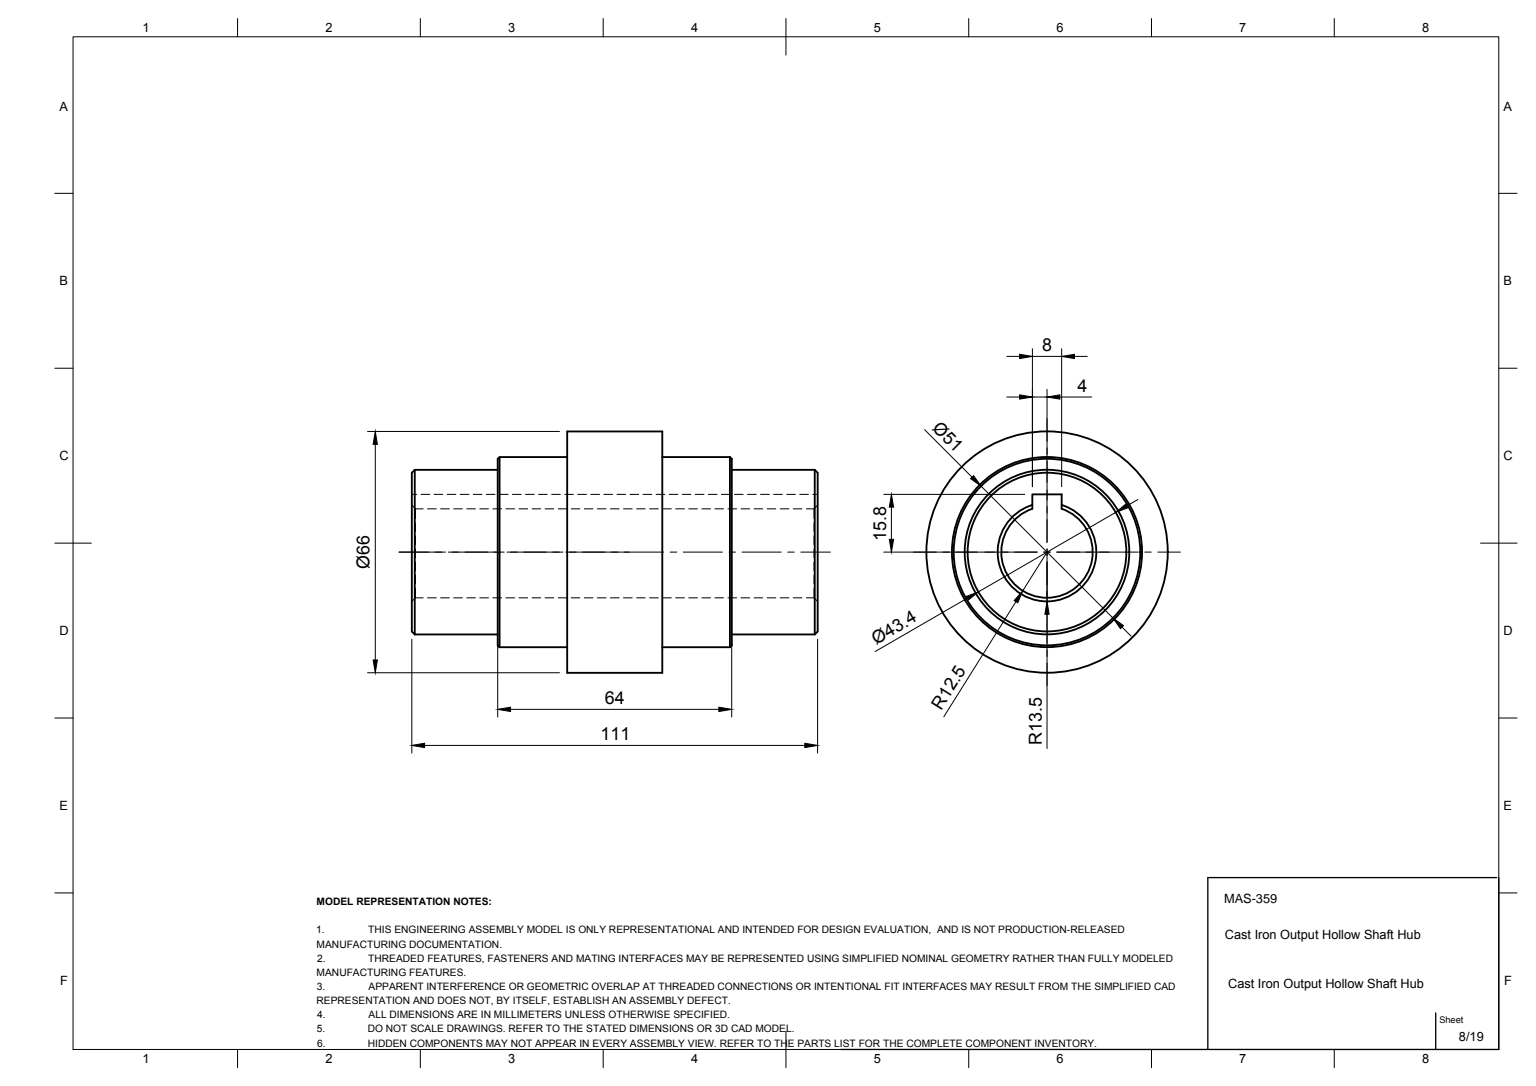
ISO-10303-21;
HEADER;
/* Generated by software containing ST-Developer
 * from STEP Tools, Inc. (www.steptools.com) 
 */

FILE_DESCRIPTION(
/* description */ (''),
/* implementation_level */ '2;1');

FILE_NAME(
/* name */ 'Cast Iron Output Hollow Shaft Hub.step',
/* time_stamp */ '2026-10-15T14:25:16-07:00',
/* author */ (''),
/* organization */ (''),
/* preprocessor_version */ 'ST-DEVELOPER v20.2',
/* originating_system */ 'Autodesk Translation Framework v15.15.0.0',
/* authorisation */ '');

FILE_SCHEMA (('AUTOMOTIVE_DESIGN { 1 0 10303 214 3 1 1 }'));
ENDSEC;

DATA;
#10=MECHANICAL_DESIGN_GEOMETRIC_PRESENTATION_REPRESENTATION('',(#328),#86429);
#262=(
BOUNDED_CURVE()
B_SPLINE_CURVE(2,(#63092,#63093,#63094),.UNSPECIFIED.,.F.,.F.)
B_SPLINE_CURVE_WITH_KNOTS((3,3),(0.,0.145078131153909),.UNSPECIFIED.)
CURVE()
GEOMETRIC_REPRESENTATION_ITEM()
RATIONAL_B_SPLINE_CURVE((1.,1.00081813630177,1.))
REPRESENTATION_ITEM('')
);
#263=(
BOUNDED_CURVE()
B_SPLINE_CURVE(2,(#63097,#63098,#63099),.UNSPECIFIED.,.F.,.F.)
B_SPLINE_CURVE_WITH_KNOTS((3,3),(0.,0.145078131153909),.UNSPECIFIED.)
CURVE()
GEOMETRIC_REPRESENTATION_ITEM()
RATIONAL_B_SPLINE_CURVE((1.,1.00081813630177,1.))
REPRESENTATION_ITEM('')
);
#264=(
BOUNDED_CURVE()
B_SPLINE_CURVE(2,(#63110,#63111,#63112),.UNSPECIFIED.,.F.,.F.)
B_SPLINE_CURVE_WITH_KNOTS((3,3),(0.,0.145078131153909),.UNSPECIFIED.)
CURVE()
GEOMETRIC_REPRESENTATION_ITEM()
RATIONAL_B_SPLINE_CURVE((1.,1.00081813630177,1.))
REPRESENTATION_ITEM('')
);
#265=(
BOUNDED_CURVE()
B_SPLINE_CURVE(2,(#63116,#63117,#63118),.UNSPECIFIED.,.F.,.F.)
B_SPLINE_CURVE_WITH_KNOTS((3,3),(0.,0.145078131153909),.UNSPECIFIED.)
CURVE()
GEOMETRIC_REPRESENTATION_ITEM()
RATIONAL_B_SPLINE_CURVE((1.,1.00081813630177,1.))
REPRESENTATION_ITEM('')
);
#292=SHAPE_REPRESENTATION_RELATIONSHIP('SRR','None',#86507,#310);
#310=ADVANCED_BREP_SHAPE_REPRESENTATION('',(#346),#86416);
#328=STYLED_ITEM('',(#86606),#346);
#346=MANIFOLD_SOLID_BREP('Body1',#15618);
#1297=CONICAL_SURFACE('',#16826,1.3,0.785398163397457);
#1298=CONICAL_SURFACE('',#16828,2.21,0.785398163397443);
#1299=CONICAL_SURFACE('',#16834,2.575,0.785398163397453);
#1300=CONICAL_SURFACE('',#16846,2.575,0.785398163397453);
#1301=CONICAL_SURFACE('',#16852,2.21,0.785398163397443);
#1302=CONICAL_SURFACE('',#16856,1.3,0.785398163397457);
#1507=CYLINDRICAL_SURFACE('',#16830,2.25);
#1508=CYLINDRICAL_SURFACE('',#16836,2.6);
#1509=CYLINDRICAL_SURFACE('',#16840,3.3);
#1510=CYLINDRICAL_SURFACE('',#16844,2.6);
#1511=CYLINDRICAL_SURFACE('',#16850,2.25);
#1512=CYLINDRICAL_SURFACE('',#16858,1.25);
#1706=FACE_BOUND('',#3993,.T.);
#1707=FACE_BOUND('',#3998,.T.);
#1708=FACE_BOUND('',#4002,.T.);
#1709=FACE_BOUND('',#4005,.T.);
#1710=FACE_BOUND('',#4009,.T.);
#1711=FACE_BOUND('',#4013,.T.);
#2198=CIRCLE('',#16824,2.17);
#2199=CIRCLE('',#16825,1.35);
#2200=CIRCLE('',#16827,1.25);
#2201=CIRCLE('',#16829,2.25);
#2202=CIRCLE('',#16831,2.25);
#2203=CIRCLE('',#16833,2.55);
#2204=CIRCLE('',#16835,2.6);
#2205=CIRCLE('',#16837,2.6);
#2206=CIRCLE('',#16839,3.3);
#2207=CIRCLE('',#16841,3.3);
#2208=CIRCLE('',#16843,2.6);
#2209=CIRCLE('',#16845,2.6);
#2210=CIRCLE('',#16847,2.55);
#2211=CIRCLE('',#16849,2.25);
#2212=CIRCLE('',#16851,2.25);
#2213=CIRCLE('',#16853,2.17);
#2214=CIRCLE('',#16855,1.35);
#2215=CIRCLE('',#16857,1.25);
#3013=FACE_OUTER_BOUND('',#3989,.T.);
#3014=FACE_OUTER_BOUND('',#3990,.T.);
#3015=FACE_OUTER_BOUND('',#3991,.T.);
#3016=FACE_OUTER_BOUND('',#3992,.T.);
#3017=FACE_OUTER_BOUND('',#3994,.T.);
#3018=FACE_OUTER_BOUND('',#3995,.T.);
#3019=FACE_OUTER_BOUND('',#3996,.T.);
#3020=FACE_OUTER_BOUND('',#3997,.T.);
#3021=FACE_OUTER_BOUND('',#3999,.T.);
#3022=FACE_OUTER_BOUND('',#4000,.T.);
#3023=FACE_OUTER_BOUND('',#4001,.T.);
#3024=FACE_OUTER_BOUND('',#4003,.T.);
#3025=FACE_OUTER_BOUND('',#4004,.T.);
#3026=FACE_OUTER_BOUND('',#4006,.T.);
#3027=FACE_OUTER_BOUND('',#4007,.T.);
#3028=FACE_OUTER_BOUND('',#4008,.T.);
#3029=FACE_OUTER_BOUND('',#4010,.T.);
#3030=FACE_OUTER_BOUND('',#4011,.T.);
#3031=FACE_OUTER_BOUND('',#4012,.T.);
#3032=FACE_OUTER_BOUND('',#4014,.T.);
#3033=FACE_OUTER_BOUND('',#4015,.T.);
#3989=EDGE_LOOP('',(#13157,#13158,#13159,#13160,#13161,#13162));
#3990=EDGE_LOOP('',(#13163,#13164,#13165,#13166));
#3991=EDGE_LOOP('',(#13167,#13168,#13169,#13170,#13171,#13172));
#3992=EDGE_LOOP('',(#13173));
#3993=EDGE_LOOP('',(#13174,#13175,#13176,#13177));
#3994=EDGE_LOOP('',(#13178,#13179,#13180,#13181));
#3995=EDGE_LOOP('',(#13182,#13183,#13184,#13185));
#3996=EDGE_LOOP('',(#13186,#13187,#13188,#13189));
#3997=EDGE_LOOP('',(#13190));
#3998=EDGE_LOOP('',(#13191));
#3999=EDGE_LOOP('',(#13192,#13193,#13194,#13195));
#4000=EDGE_LOOP('',(#13196,#13197,#13198,#13199));
#4001=EDGE_LOOP('',(#13200));
#4002=EDGE_LOOP('',(#13201));
#4003=EDGE_LOOP('',(#13202,#13203,#13204,#13205));
#4004=EDGE_LOOP('',(#13206));
#4005=EDGE_LOOP('',(#13207));
#4006=EDGE_LOOP('',(#13208,#13209,#13210,#13211));
#4007=EDGE_LOOP('',(#13212,#13213,#13214,#13215));
#4008=EDGE_LOOP('',(#13216));
#4009=EDGE_LOOP('',(#13217));
#4010=EDGE_LOOP('',(#13218,#13219,#13220,#13221));
#4011=EDGE_LOOP('',(#13222,#13223,#13224,#13225));
#4012=EDGE_LOOP('',(#13226));
#4013=EDGE_LOOP('',(#13227,#13228,#13229,#13230));
#4014=EDGE_LOOP('',(#13231,#13232,#13233,#13234));
#4015=EDGE_LOOP('',(#13235,#13236,#13237,#13238));
#4949=LINE('',#63086,#5809);
#4950=LINE('',#63088,#5810);
#4951=LINE('',#63090,#5811);
#4952=LINE('',#63096,#5812);
#4953=LINE('',#63102,#5813);
#4954=LINE('',#63104,#5814);
#4955=LINE('',#63105,#5815);
#4956=LINE('',#63108,#5816);
#4957=LINE('',#63114,#5817);
#4958=LINE('',#63119,#5818);
#4959=LINE('',#63129,#5819);
#4960=LINE('',#63133,#5820);
#4961=LINE('',#63140,#5821);
#4962=LINE('',#63144,#5822);
#4963=LINE('',#63151,#5823);
#4964=LINE('',#63158,#5824);
#4965=LINE('',#63161,#5825);
#4966=LINE('',#63169,#5826);
#4967=LINE('',#63172,#5827);
#5809=VECTOR('',#19936,1.);
#5810=VECTOR('',#19937,1.);
#5811=VECTOR('',#19938,1.);
#5812=VECTOR('',#19939,1.);
#5813=VECTOR('',#19942,1.);
#5814=VECTOR('',#19943,1.);
#5815=VECTOR('',#19944,1.);
#5816=VECTOR('',#19947,1.);
#5817=VECTOR('',#19948,1.);
#5818=VECTOR('',#19949,1.);
#5819=VECTOR('',#19964,2.21);
#5820=VECTOR('',#19969,2.25);
#5821=VECTOR('',#19978,2.575);
#5822=VECTOR('',#19983,2.6);
#5823=VECTOR('',#19992,3.3);
#5824=VECTOR('',#20001,2.6);
#5825=VECTOR('',#20004,2.575);
#5826=VECTOR('',#20015,2.25);
#5827=VECTOR('',#20018,2.21);
#7082=VERTEX_POINT('',#63084);
#7083=VERTEX_POINT('',#63085);
#7084=VERTEX_POINT('',#63087);
#7085=VERTEX_POINT('',#63089);
#7086=VERTEX_POINT('',#63091);
#7087=VERTEX_POINT('',#63095);
#7088=VERTEX_POINT('',#63101);
#7089=VERTEX_POINT('',#63103);
#7090=VERTEX_POINT('',#63107);
#7091=VERTEX_POINT('',#63109);
#7092=VERTEX_POINT('',#63113);
#7093=VERTEX_POINT('',#63115);
#7094=VERTEX_POINT('',#63121);
#7095=VERTEX_POINT('',#63127);
#7096=VERTEX_POINT('',#63131);
#7097=VERTEX_POINT('',#63135);
#7098=VERTEX_POINT('',#63138);
#7099=VERTEX_POINT('',#63142);
#7100=VERTEX_POINT('',#63146);
#7101=VERTEX_POINT('',#63149);
#7102=VERTEX_POINT('',#63153);
#7103=VERTEX_POINT('',#63156);
#7104=VERTEX_POINT('',#63160);
#7105=VERTEX_POINT('',#63164);
#7106=VERTEX_POINT('',#63167);
#7107=VERTEX_POINT('',#63171);
#9200=EDGE_CURVE('',#7082,#7083,#4949,.T.);
#9201=EDGE_CURVE('',#7082,#7084,#4950,.T.);
#9202=EDGE_CURVE('',#7085,#7084,#4951,.T.);
#9203=EDGE_CURVE('',#7086,#7085,#262,.T.);
#9204=EDGE_CURVE('',#7087,#7086,#4952,.T.);
#9205=EDGE_CURVE('',#7083,#7087,#263,.T.);
#9206=EDGE_CURVE('',#7088,#7082,#4953,.T.);
#9207=EDGE_CURVE('',#7089,#7088,#4954,.T.);
#9208=EDGE_CURVE('',#7084,#7089,#4955,.T.);
#9209=EDGE_CURVE('',#7090,#7088,#4956,.T.);
#9210=EDGE_CURVE('',#7091,#7090,#264,.T.);
#9211=EDGE_CURVE('',#7092,#7091,#4957,.T.);
#9212=EDGE_CURVE('',#7093,#7092,#265,.T.);
#9213=EDGE_CURVE('',#7089,#7093,#4958,.T.);
#9214=EDGE_CURVE('',#7094,#7094,#2198,.T.);
#9215=EDGE_CURVE('',#7083,#7090,#2199,.T.);
#9216=EDGE_CURVE('',#7087,#7091,#2200,.T.);
#9217=EDGE_CURVE('',#7095,#7095,#2201,.T.);
#9218=EDGE_CURVE('',#7095,#7094,#4959,.T.);
#9219=EDGE_CURVE('',#7096,#7096,#2202,.T.);
#9220=EDGE_CURVE('',#7096,#7095,#4960,.T.);
#9221=EDGE_CURVE('',#7097,#7097,#2203,.T.);
#9222=EDGE_CURVE('',#7098,#7098,#2204,.T.);
#9223=EDGE_CURVE('',#7098,#7097,#4961,.T.);
#9224=EDGE_CURVE('',#7099,#7099,#2205,.T.);
#9225=EDGE_CURVE('',#7099,#7098,#4962,.T.);
#9226=EDGE_CURVE('',#7100,#7100,#2206,.T.);
#9227=EDGE_CURVE('',#7101,#7101,#2207,.T.);
#9228=EDGE_CURVE('',#7101,#7100,#4963,.T.);
#9229=EDGE_CURVE('',#7102,#7102,#2208,.T.);
#9230=EDGE_CURVE('',#7103,#7103,#2209,.T.);
#9231=EDGE_CURVE('',#7103,#7102,#4964,.T.);
#9232=EDGE_CURVE('',#7103,#7104,#4965,.T.);
#9233=EDGE_CURVE('',#7104,#7104,#2210,.T.);
#9234=EDGE_CURVE('',#7105,#7105,#2211,.T.);
#9235=EDGE_CURVE('',#7106,#7106,#2212,.T.);
#9236=EDGE_CURVE('',#7106,#7105,#4966,.T.);
#9237=EDGE_CURVE('',#7106,#7107,#4967,.T.);
#9238=EDGE_CURVE('',#7107,#7107,#2213,.T.);
#9239=EDGE_CURVE('',#7085,#7093,#2214,.T.);
#9240=EDGE_CURVE('',#7086,#7092,#2215,.T.);
#13157=ORIENTED_EDGE('',*,*,#9200,.F.);
#13158=ORIENTED_EDGE('',*,*,#9201,.T.);
#13159=ORIENTED_EDGE('',*,*,#9202,.F.);
#13160=ORIENTED_EDGE('',*,*,#9203,.F.);
#13161=ORIENTED_EDGE('',*,*,#9204,.F.);
#13162=ORIENTED_EDGE('',*,*,#9205,.F.);
#13163=ORIENTED_EDGE('',*,*,#9206,.F.);
#13164=ORIENTED_EDGE('',*,*,#9207,.F.);
#13165=ORIENTED_EDGE('',*,*,#9208,.F.);
#13166=ORIENTED_EDGE('',*,*,#9201,.F.);
#13167=ORIENTED_EDGE('',*,*,#9209,.F.);
#13168=ORIENTED_EDGE('',*,*,#9210,.F.);
#13169=ORIENTED_EDGE('',*,*,#9211,.F.);
#13170=ORIENTED_EDGE('',*,*,#9212,.F.);
#13171=ORIENTED_EDGE('',*,*,#9213,.F.);
#13172=ORIENTED_EDGE('',*,*,#9207,.T.);
#13173=ORIENTED_EDGE('',*,*,#9214,.F.);
#13174=ORIENTED_EDGE('',*,*,#9209,.T.);
#13175=ORIENTED_EDGE('',*,*,#9206,.T.);
#13176=ORIENTED_EDGE('',*,*,#9200,.T.);
#13177=ORIENTED_EDGE('',*,*,#9215,.T.);
#13178=ORIENTED_EDGE('',*,*,#9210,.T.);
#13179=ORIENTED_EDGE('',*,*,#9215,.F.);
#13180=ORIENTED_EDGE('',*,*,#9205,.T.);
#13181=ORIENTED_EDGE('',*,*,#9216,.T.);
#13182=ORIENTED_EDGE('',*,*,#9217,.F.);
#13183=ORIENTED_EDGE('',*,*,#9218,.T.);
#13184=ORIENTED_EDGE('',*,*,#9214,.T.);
#13185=ORIENTED_EDGE('',*,*,#9218,.F.);
#13186=ORIENTED_EDGE('',*,*,#9219,.F.);
#13187=ORIENTED_EDGE('',*,*,#9220,.T.);
#13188=ORIENTED_EDGE('',*,*,#9217,.T.);
#13189=ORIENTED_EDGE('',*,*,#9220,.F.);
#13190=ORIENTED_EDGE('',*,*,#9221,.F.);
#13191=ORIENTED_EDGE('',*,*,#9219,.T.);
#13192=ORIENTED_EDGE('',*,*,#9222,.F.);
#13193=ORIENTED_EDGE('',*,*,#9223,.T.);
#13194=ORIENTED_EDGE('',*,*,#9221,.T.);
#13195=ORIENTED_EDGE('',*,*,#9223,.F.);
#13196=ORIENTED_EDGE('',*,*,#9224,.F.);
#13197=ORIENTED_EDGE('',*,*,#9225,.T.);
#13198=ORIENTED_EDGE('',*,*,#9222,.T.);
#13199=ORIENTED_EDGE('',*,*,#9225,.F.);
#13200=ORIENTED_EDGE('',*,*,#9226,.F.);
#13201=ORIENTED_EDGE('',*,*,#9224,.T.);
#13202=ORIENTED_EDGE('',*,*,#9227,.F.);
#13203=ORIENTED_EDGE('',*,*,#9228,.T.);
#13204=ORIENTED_EDGE('',*,*,#9226,.T.);
#13205=ORIENTED_EDGE('',*,*,#9228,.F.);
#13206=ORIENTED_EDGE('',*,*,#9227,.T.);
#13207=ORIENTED_EDGE('',*,*,#9229,.F.);
#13208=ORIENTED_EDGE('',*,*,#9230,.F.);
#13209=ORIENTED_EDGE('',*,*,#9231,.T.);
#13210=ORIENTED_EDGE('',*,*,#9229,.T.);
#13211=ORIENTED_EDGE('',*,*,#9231,.F.);
#13212=ORIENTED_EDGE('',*,*,#9230,.T.);
#13213=ORIENTED_EDGE('',*,*,#9232,.T.);
#13214=ORIENTED_EDGE('',*,*,#9233,.F.);
#13215=ORIENTED_EDGE('',*,*,#9232,.F.);
#13216=ORIENTED_EDGE('',*,*,#9233,.T.);
#13217=ORIENTED_EDGE('',*,*,#9234,.F.);
#13218=ORIENTED_EDGE('',*,*,#9235,.F.);
#13219=ORIENTED_EDGE('',*,*,#9236,.T.);
#13220=ORIENTED_EDGE('',*,*,#9234,.T.);
#13221=ORIENTED_EDGE('',*,*,#9236,.F.);
#13222=ORIENTED_EDGE('',*,*,#9235,.T.);
#13223=ORIENTED_EDGE('',*,*,#9237,.T.);
#13224=ORIENTED_EDGE('',*,*,#9238,.F.);
#13225=ORIENTED_EDGE('',*,*,#9237,.F.);
#13226=ORIENTED_EDGE('',*,*,#9238,.T.);
#13227=ORIENTED_EDGE('',*,*,#9213,.T.);
#13228=ORIENTED_EDGE('',*,*,#9239,.F.);
#13229=ORIENTED_EDGE('',*,*,#9202,.T.);
#13230=ORIENTED_EDGE('',*,*,#9208,.T.);
#13231=ORIENTED_EDGE('',*,*,#9212,.T.);
#13232=ORIENTED_EDGE('',*,*,#9240,.F.);
#13233=ORIENTED_EDGE('',*,*,#9203,.T.);
#13234=ORIENTED_EDGE('',*,*,#9239,.T.);
#13235=ORIENTED_EDGE('',*,*,#9211,.T.);
#13236=ORIENTED_EDGE('',*,*,#9216,.F.);
#13237=ORIENTED_EDGE('',*,*,#9204,.T.);
#13238=ORIENTED_EDGE('',*,*,#9240,.T.);
#14656=PLANE('',#16820);
#14657=PLANE('',#16821);
#14658=PLANE('',#16822);
#14659=PLANE('',#16823);
#14660=PLANE('',#16832);
#14661=PLANE('',#16838);
#14662=PLANE('',#16842);
#14663=PLANE('',#16848);
#14664=PLANE('',#16854);
#15369=ADVANCED_FACE('',(#3013),#14656,.F.);
#15370=ADVANCED_FACE('',(#3014),#14657,.F.);
#15371=ADVANCED_FACE('',(#3015),#14658,.F.);
#15372=ADVANCED_FACE('',(#3016,#1706),#14659,.T.);
#15373=ADVANCED_FACE('',(#3017),#1297,.F.);
#15374=ADVANCED_FACE('',(#3018),#1298,.T.);
#15375=ADVANCED_FACE('',(#3019),#1507,.T.);
#15376=ADVANCED_FACE('',(#3020,#1707),#14660,.T.);
#15377=ADVANCED_FACE('',(#3021),#1299,.T.);
#15378=ADVANCED_FACE('',(#3022),#1508,.T.);
#15379=ADVANCED_FACE('',(#3023,#1708),#14661,.T.);
#15380=ADVANCED_FACE('',(#3024),#1509,.T.);
#15381=ADVANCED_FACE('',(#3025,#1709),#14662,.T.);
#15382=ADVANCED_FACE('',(#3026),#1510,.T.);
#15383=ADVANCED_FACE('',(#3027),#1300,.T.);
#15384=ADVANCED_FACE('',(#3028,#1710),#14663,.T.);
#15385=ADVANCED_FACE('',(#3029),#1511,.T.);
#15386=ADVANCED_FACE('',(#3030),#1301,.T.);
#15387=ADVANCED_FACE('',(#3031,#1711),#14664,.T.);
#15388=ADVANCED_FACE('',(#3032),#1302,.F.);
#15389=ADVANCED_FACE('',(#3033),#1512,.F.);
#15618=CLOSED_SHELL('',(#15369,#15370,#15371,#15372,#15373,#15374,#15375,
#15376,#15377,#15378,#15379,#15380,#15381,#15382,#15383,#15384,#15385,#15386,
#15387,#15388,#15389));
#16819=AXIS2_PLACEMENT_3D('',#63082,#19932,#19933);
#16820=AXIS2_PLACEMENT_3D('',#63083,#19934,#19935);
#16821=AXIS2_PLACEMENT_3D('',#63100,#19940,#19941);
#16822=AXIS2_PLACEMENT_3D('',#63106,#19945,#19946);
#16823=AXIS2_PLACEMENT_3D('',#63120,#19950,#19951);
#16824=AXIS2_PLACEMENT_3D('',#63122,#19952,#19953);
#16825=AXIS2_PLACEMENT_3D('',#63123,#19954,#19955);
#16826=AXIS2_PLACEMENT_3D('',#63124,#19956,#19957);
#16827=AXIS2_PLACEMENT_3D('',#63125,#19958,#19959);
#16828=AXIS2_PLACEMENT_3D('',#63126,#19960,#19961);
#16829=AXIS2_PLACEMENT_3D('',#63128,#19962,#19963);
#16830=AXIS2_PLACEMENT_3D('',#63130,#19965,#19966);
#16831=AXIS2_PLACEMENT_3D('',#63132,#19967,#19968);
#16832=AXIS2_PLACEMENT_3D('',#63134,#19970,#19971);
#16833=AXIS2_PLACEMENT_3D('',#63136,#19972,#19973);
#16834=AXIS2_PLACEMENT_3D('',#63137,#19974,#19975);
#16835=AXIS2_PLACEMENT_3D('',#63139,#19976,#19977);
#16836=AXIS2_PLACEMENT_3D('',#63141,#19979,#19980);
#16837=AXIS2_PLACEMENT_3D('',#63143,#19981,#19982);
#16838=AXIS2_PLACEMENT_3D('',#63145,#19984,#19985);
#16839=AXIS2_PLACEMENT_3D('',#63147,#19986,#19987);
#16840=AXIS2_PLACEMENT_3D('',#63148,#19988,#19989);
#16841=AXIS2_PLACEMENT_3D('',#63150,#19990,#19991);
#16842=AXIS2_PLACEMENT_3D('',#63152,#19993,#19994);
#16843=AXIS2_PLACEMENT_3D('',#63154,#19995,#19996);
#16844=AXIS2_PLACEMENT_3D('',#63155,#19997,#19998);
#16845=AXIS2_PLACEMENT_3D('',#63157,#19999,#20000);
#16846=AXIS2_PLACEMENT_3D('',#63159,#20002,#20003);
#16847=AXIS2_PLACEMENT_3D('',#63162,#20005,#20006);
#16848=AXIS2_PLACEMENT_3D('',#63163,#20007,#20008);
#16849=AXIS2_PLACEMENT_3D('',#63165,#20009,#20010);
#16850=AXIS2_PLACEMENT_3D('',#63166,#20011,#20012);
#16851=AXIS2_PLACEMENT_3D('',#63168,#20013,#20014);
#16852=AXIS2_PLACEMENT_3D('',#63170,#20016,#20017);
#16853=AXIS2_PLACEMENT_3D('',#63173,#20019,#20020);
#16854=AXIS2_PLACEMENT_3D('',#63174,#20021,#20022);
#16855=AXIS2_PLACEMENT_3D('',#63175,#20023,#20024);
#16856=AXIS2_PLACEMENT_3D('',#63176,#20025,#20026);
#16857=AXIS2_PLACEMENT_3D('',#63177,#20027,#20028);
#16858=AXIS2_PLACEMENT_3D('',#63178,#20029,#20030);
#19932=DIRECTION('axis',(0.,0.,1.));
#19933=DIRECTION('refdir',(1.,0.,0.));
#19934=DIRECTION('center_axis',(1.,0.,0.));
#19935=DIRECTION('ref_axis',(0.,0.,-1.));
#19936=DIRECTION('',(0.,0.,-1.));
#19937=DIRECTION('',(0.,1.,0.));
#19938=DIRECTION('',(0.,0.,1.));
#19939=DIRECTION('',(0.,1.,0.));
#19940=DIRECTION('center_axis',(0.,0.,1.));
#19941=DIRECTION('ref_axis',(1.,0.,0.));
#19942=DIRECTION('',(1.,0.,0.));
#19943=DIRECTION('',(0.,-1.,0.));
#19944=DIRECTION('',(-1.,0.,0.));
#19945=DIRECTION('center_axis',(-1.,0.,0.));
#19946=DIRECTION('ref_axis',(0.,0.,1.));
#19947=DIRECTION('',(0.,0.,1.));
#19948=DIRECTION('',(0.,-1.,0.));
#19949=DIRECTION('',(0.,0.,-1.));
#19950=DIRECTION('center_axis',(0.,-1.,0.));
#19951=DIRECTION('ref_axis',(0.,0.,-1.));
#19952=DIRECTION('center_axis',(0.,1.,0.));
#19953=DIRECTION('ref_axis',(1.,0.,0.));
#19954=DIRECTION('center_axis',(0.,1.,0.));
#19955=DIRECTION('ref_axis',(1.,0.,0.));
#19956=DIRECTION('center_axis',(0.,-1.,0.));
#19957=DIRECTION('ref_axis',(-1.22464679914735E-16,0.,-1.));
#19958=DIRECTION('center_axis',(0.,1.,0.));
#19959=DIRECTION('ref_axis',(1.,0.,0.));
#19960=DIRECTION('center_axis',(0.,1.,0.));
#19961=DIRECTION('ref_axis',(0.,0.,1.));
#19962=DIRECTION('center_axis',(0.,1.,0.));
#19963=DIRECTION('ref_axis',(1.,0.,0.));
#19964=DIRECTION('',(8.65956056235489E-17,-0.707106781186551,0.707106781186544));
#19965=DIRECTION('center_axis',(0.,1.,0.));
#19966=DIRECTION('ref_axis',(0.,0.,1.));
#19967=DIRECTION('center_axis',(0.,1.,0.));
#19968=DIRECTION('ref_axis',(1.,0.,0.));
#19969=DIRECTION('',(0.,-1.,0.));
#19970=DIRECTION('center_axis',(0.,-1.,0.));
#19971=DIRECTION('ref_axis',(0.,0.,-1.));
#19972=DIRECTION('center_axis',(0.,1.,0.));
#19973=DIRECTION('ref_axis',(1.,0.,0.));
#19974=DIRECTION('center_axis',(0.,1.,0.));
#19975=DIRECTION('ref_axis',(0.,0.,1.));
#19976=DIRECTION('center_axis',(0.,1.,0.));
#19977=DIRECTION('ref_axis',(1.,0.,0.));
#19978=DIRECTION('',(8.65956056235497E-17,-0.707106781186544,0.707106781186551));
#19979=DIRECTION('center_axis',(0.,1.,0.));
#19980=DIRECTION('ref_axis',(0.,0.,1.));
#19981=DIRECTION('center_axis',(0.,1.,0.));
#19982=DIRECTION('ref_axis',(1.,0.,0.));
#19983=DIRECTION('',(0.,-1.,0.));
#19984=DIRECTION('center_axis',(0.,-1.,0.));
#19985=DIRECTION('ref_axis',(0.,0.,-1.));
#19986=DIRECTION('center_axis',(0.,1.,0.));
#19987=DIRECTION('ref_axis',(1.,0.,0.));
#19988=DIRECTION('center_axis',(0.,1.,0.));
#19989=DIRECTION('ref_axis',(0.,0.,1.));
#19990=DIRECTION('center_axis',(0.,1.,0.));
#19991=DIRECTION('ref_axis',(1.,0.,0.));
#19992=DIRECTION('',(0.,-1.,0.));
#19993=DIRECTION('center_axis',(0.,1.,0.));
#19994=DIRECTION('ref_axis',(0.,0.,1.));
#19995=DIRECTION('center_axis',(0.,1.,0.));
#19996=DIRECTION('ref_axis',(1.,0.,0.));
#19997=DIRECTION('center_axis',(0.,1.,0.));
#19998=DIRECTION('ref_axis',(0.,0.,1.));
#19999=DIRECTION('center_axis',(0.,1.,0.));
#20000=DIRECTION('ref_axis',(1.,0.,0.));
#20001=DIRECTION('',(0.,-1.,0.));
#20002=DIRECTION('center_axis',(0.,-1.,0.));
#20003=DIRECTION('ref_axis',(0.,0.,1.));
#20004=DIRECTION('',(-8.65956056235497E-17,0.707106781186544,0.707106781186551));
#20005=DIRECTION('center_axis',(0.,1.,0.));
#20006=DIRECTION('ref_axis',(1.,0.,0.));
#20007=DIRECTION('center_axis',(0.,1.,0.));
#20008=DIRECTION('ref_axis',(0.,0.,1.));
#20009=DIRECTION('center_axis',(0.,1.,0.));
#20010=DIRECTION('ref_axis',(1.,0.,0.));
#20011=DIRECTION('center_axis',(0.,1.,0.));
#20012=DIRECTION('ref_axis',(0.,0.,1.));
#20013=DIRECTION('center_axis',(0.,1.,0.));
#20014=DIRECTION('ref_axis',(1.,0.,0.));
#20015=DIRECTION('',(0.,-1.,0.));
#20016=DIRECTION('center_axis',(0.,-1.,0.));
#20017=DIRECTION('ref_axis',(0.,0.,1.));
#20018=DIRECTION('',(-8.65956056235489E-17,0.707106781186551,0.707106781186544));
#20019=DIRECTION('center_axis',(0.,1.,0.));
#20020=DIRECTION('ref_axis',(1.,0.,0.));
#20021=DIRECTION('center_axis',(0.,1.,0.));
#20022=DIRECTION('ref_axis',(0.,0.,1.));
#20023=DIRECTION('center_axis',(0.,1.,0.));
#20024=DIRECTION('ref_axis',(1.,0.,0.));
#20025=DIRECTION('center_axis',(0.,1.,0.));
#20026=DIRECTION('ref_axis',(-1.22464679914735E-16,0.,-1.));
#20027=DIRECTION('center_axis',(0.,1.,0.));
#20028=DIRECTION('ref_axis',(1.,0.,0.));
#20029=DIRECTION('center_axis',(0.,1.,0.));
#20030=DIRECTION('ref_axis',(-1.22464679914735E-16,0.,-1.));
#63082=CARTESIAN_POINT('',(0.,0.,0.));
#63083=CARTESIAN_POINT('Origin',(0.4,0.,8.78));
#63084=CARTESIAN_POINT('',(0.4,-5.55,8.78));
#63085=CARTESIAN_POINT('',(0.4,-5.55,8.48937969582276));
#63086=CARTESIAN_POINT('',(0.4,-5.55,9.075));
#63087=CARTESIAN_POINT('',(0.4,5.55,8.78));
#63088=CARTESIAN_POINT('',(0.4,0.,8.78));
#63089=CARTESIAN_POINT('',(0.4,5.55,8.48937969582276));
#63090=CARTESIAN_POINT('',(0.4,5.55,8.665));
#63091=CARTESIAN_POINT('',(0.4,5.45,8.3842719282327));
#63092=CARTESIAN_POINT('Ctrl Pts',(0.4,5.45,8.3842719282327));
#63093=CARTESIAN_POINT('Ctrl Pts',(0.4,5.49787545330696,8.43480450880564));
#63094=CARTESIAN_POINT('Ctrl Pts',(0.4,5.55,8.48937969582276));
#63095=CARTESIAN_POINT('',(0.4,-5.45,8.3842719282327));
#63096=CARTESIAN_POINT('',(0.4,0.,8.3842719282327));
#63097=CARTESIAN_POINT('Ctrl Pts',(0.4,-5.55,8.48937969582276));
#63098=CARTESIAN_POINT('Ctrl Pts',(0.4,-5.49787545330696,8.43480450880564));
#63099=CARTESIAN_POINT('Ctrl Pts',(0.4,-5.45,8.3842719282327));
#63100=CARTESIAN_POINT('Origin',(-0.4,0.,8.78));
#63101=CARTESIAN_POINT('',(-0.4,-5.55,8.78));
#63102=CARTESIAN_POINT('',(-0.2,-5.55,8.78));
#63103=CARTESIAN_POINT('',(-0.4,5.55,8.78));
#63104=CARTESIAN_POINT('',(-0.4,0.,8.78));
#63105=CARTESIAN_POINT('',(-0.2,5.55,8.78));
#63106=CARTESIAN_POINT('Origin',(-0.4,0.,7.2));
#63107=CARTESIAN_POINT('',(-0.4,-5.55,8.48937969582276));
#63108=CARTESIAN_POINT('',(-0.4,-5.55,8.285));
#63109=CARTESIAN_POINT('',(-0.4,-5.45,8.3842719282327));
#63110=CARTESIAN_POINT('Ctrl Pts',(-0.4,-5.45,8.3842719282327));
#63111=CARTESIAN_POINT('Ctrl Pts',(-0.4,-5.49787545330696,8.43480450880564));
#63112=CARTESIAN_POINT('Ctrl Pts',(-0.4,-5.55,8.48937969582276));
#63113=CARTESIAN_POINT('',(-0.4,5.45,8.3842719282327));
#63114=CARTESIAN_POINT('',(-0.4,0.,8.3842719282327));
#63115=CARTESIAN_POINT('',(-0.4,5.55,8.48937969582276));
#63116=CARTESIAN_POINT('Ctrl Pts',(-0.4,5.55,8.48937969582276));
#63117=CARTESIAN_POINT('Ctrl Pts',(-0.4,5.49787545330696,8.43480450880564));
#63118=CARTESIAN_POINT('Ctrl Pts',(-0.4,5.45,8.3842719282327));
#63119=CARTESIAN_POINT('',(-0.4,5.55,7.875));
#63120=CARTESIAN_POINT('Origin',(0.,-5.55,9.37));
#63121=CARTESIAN_POINT('',(-2.65748355414976E-16,-5.55,5.03));
#63122=CARTESIAN_POINT('Origin',(0.,-5.55,7.2));
#63123=CARTESIAN_POINT('Origin',(0.,-5.55,7.2));
#63124=CARTESIAN_POINT('Origin',(0.,-5.5,7.2));
#63125=CARTESIAN_POINT('Origin',(0.,-5.45,7.2));
#63126=CARTESIAN_POINT('Origin',(0.,-5.51,7.2));
#63127=CARTESIAN_POINT('',(-2.75545529808154E-16,-5.47,4.95));
#63128=CARTESIAN_POINT('Origin',(0.,-5.47,7.2));
#63129=CARTESIAN_POINT('',(-2.70646942611565E-16,-5.51,4.99));
#63130=CARTESIAN_POINT('Origin',(0.,-4.335,7.2));
#63131=CARTESIAN_POINT('',(-2.75545529808154E-16,-3.2,4.95));
#63132=CARTESIAN_POINT('Origin',(0.,-3.2,7.2));
#63133=CARTESIAN_POINT('',(-2.75545529808154E-16,-4.335,4.95));
#63134=CARTESIAN_POINT('Origin',(0.,-3.2,9.75));
#63135=CARTESIAN_POINT('',(-3.12284933782575E-16,-3.2,4.65));
#63136=CARTESIAN_POINT('Origin',(0.,-3.2,7.2));
#63137=CARTESIAN_POINT('Origin',(0.,-3.175,7.2));
#63138=CARTESIAN_POINT('',(-3.18408167778312E-16,-3.15,4.6));
#63139=CARTESIAN_POINT('Origin',(0.,-3.15,7.2));
#63140=CARTESIAN_POINT('',(-3.15346550780443E-16,-3.175,4.625));
#63141=CARTESIAN_POINT('Origin',(0.,-2.225,7.2));
#63142=CARTESIAN_POINT('',(-3.18408167778312E-16,-1.3,4.6));
#63143=CARTESIAN_POINT('Origin',(0.,-1.3,7.2));
#63144=CARTESIAN_POINT('',(-3.18408167778312E-16,-2.225,4.6));
#63145=CARTESIAN_POINT('Origin',(0.,-1.3,10.5));
#63146=CARTESIAN_POINT('',(-4.04133443718627E-16,-1.3,3.9));
#63147=CARTESIAN_POINT('Origin',(0.,-1.3,7.2));
#63148=CARTESIAN_POINT('Origin',(0.,0.,7.2));
#63149=CARTESIAN_POINT('',(-4.04133443718627E-16,1.3,3.9));
#63150=CARTESIAN_POINT('Origin',(0.,1.3,7.2));
#63151=CARTESIAN_POINT('',(-4.04133443718627E-16,0.,3.9));
#63152=CARTESIAN_POINT('Origin',(0.,1.3,9.8));
#63153=CARTESIAN_POINT('',(-3.18408167778312E-16,1.3,4.6));
#63154=CARTESIAN_POINT('Origin',(0.,1.3,7.2));
#63155=CARTESIAN_POINT('Origin',(0.,2.225,7.2));
#63156=CARTESIAN_POINT('',(-3.18408167778312E-16,3.15,4.6));
#63157=CARTESIAN_POINT('Origin',(0.,3.15,7.2));
#63158=CARTESIAN_POINT('',(-3.18408167778312E-16,2.225,4.6));
#63159=CARTESIAN_POINT('Origin',(0.,3.175,7.2));
#63160=CARTESIAN_POINT('',(-3.12284933782575E-16,3.2,4.65));
#63161=CARTESIAN_POINT('',(3.15346550780443E-16,3.175,4.625));
#63162=CARTESIAN_POINT('Origin',(0.,3.2,7.2));
#63163=CARTESIAN_POINT('Origin',(0.,3.2,9.45));
#63164=CARTESIAN_POINT('',(-2.75545529808154E-16,3.2,4.95));
#63165=CARTESIAN_POINT('Origin',(0.,3.2,7.2));
#63166=CARTESIAN_POINT('Origin',(0.,4.335,7.2));
#63167=CARTESIAN_POINT('',(-2.75545529808154E-16,5.47,4.95));
#63168=CARTESIAN_POINT('Origin',(0.,5.47,7.2));
#63169=CARTESIAN_POINT('',(-2.75545529808154E-16,4.335,4.95));
#63170=CARTESIAN_POINT('Origin',(0.,5.51,7.2));
#63171=CARTESIAN_POINT('',(-2.65748355414976E-16,5.55,5.03));
#63172=CARTESIAN_POINT('',(2.70646942611565E-16,5.51,4.99));
#63173=CARTESIAN_POINT('Origin',(0.,5.55,7.2));
#63174=CARTESIAN_POINT('Origin',(0.,5.55,8.55));
#63175=CARTESIAN_POINT('Origin',(0.,5.55,7.2));
#63176=CARTESIAN_POINT('Origin',(0.,5.5,7.2));
#63177=CARTESIAN_POINT('Origin',(0.,5.45,7.2));
#63178=CARTESIAN_POINT('Origin',(0.,0.,7.2));
#86396=UNCERTAINTY_MEASURE_WITH_UNIT(LENGTH_MEASURE(0.001),#86430,
'DISTANCE_ACCURACY_VALUE',
'Maximum model space distance between geometric entities at asserted c
onnectivities');
#86409=UNCERTAINTY_MEASURE_WITH_UNIT(LENGTH_MEASURE(0.001),#86430,
'DISTANCE_ACCURACY_VALUE',
'Maximum model space distance between geometric entities at asserted c
onnectivities');
#86416=(
GEOMETRIC_REPRESENTATION_CONTEXT(3)
GLOBAL_UNCERTAINTY_ASSIGNED_CONTEXT((#86396))
GLOBAL_UNIT_ASSIGNED_CONTEXT((#86430,#86432,#86433))
REPRESENTATION_CONTEXT('','3D')
);
#86429=(
GEOMETRIC_REPRESENTATION_CONTEXT(3)
GLOBAL_UNCERTAINTY_ASSIGNED_CONTEXT((#86409))
GLOBAL_UNIT_ASSIGNED_CONTEXT((#86430,#86432,#86433))
REPRESENTATION_CONTEXT('','3D')
);
#86430=(
LENGTH_UNIT()
NAMED_UNIT(*)
SI_UNIT(.CENTI.,.METRE.)
);
#86432=(
NAMED_UNIT(*)
PLANE_ANGLE_UNIT()
SI_UNIT($,.RADIAN.)
);
#86433=(
NAMED_UNIT(*)
SI_UNIT($,.STERADIAN.)
SOLID_ANGLE_UNIT()
);
#86440=SHAPE_DEFINITION_REPRESENTATION(#86459,#86507);
#86459=PRODUCT_DEFINITION_SHAPE('',$,#86527);
#86507=SHAPE_REPRESENTATION('',(#16819),#86416);
#86520=PRODUCT_DEFINITION_CONTEXT('part definition',#86579,'design');
#86527=PRODUCT_DEFINITION('Cast Iron Output Hollow Shaft Hub',
'Cast Iron Output Hollow Shaft Hub',#86546,#86520);
#86546=PRODUCT_DEFINITION_FORMATION('',$,#86587);
#86579=APPLICATION_CONTEXT(
'Core Data for Automotive Mechanical Design Process');
#86580=PRODUCT_CONTEXT('part definition',#86579,'mechanical');
#86587=PRODUCT('Cast Iron Output Hollow Shaft Hub',
'Cast Iron Output Hollow Shaft Hub',$,(#86580));
#86606=PRESENTATION_STYLE_ASSIGNMENT((#86624));
#86624=SURFACE_STYLE_USAGE(.BOTH.,#86642);
#86642=SURFACE_SIDE_STYLE('',(#86660));
#86660=SURFACE_STYLE_FILL_AREA(#86678);
#86678=FILL_AREA_STYLE('Opaque(128,131,135)',(#86696));
#86696=FILL_AREA_STYLE_COLOUR('Opaque(128,131,135)',#86714);
#86714=COLOUR_RGB('Opaque(128,131,135)', 0.08235294, 0.09019608, 0.10196078);
ENDSEC;
END-ISO-10303-21;
